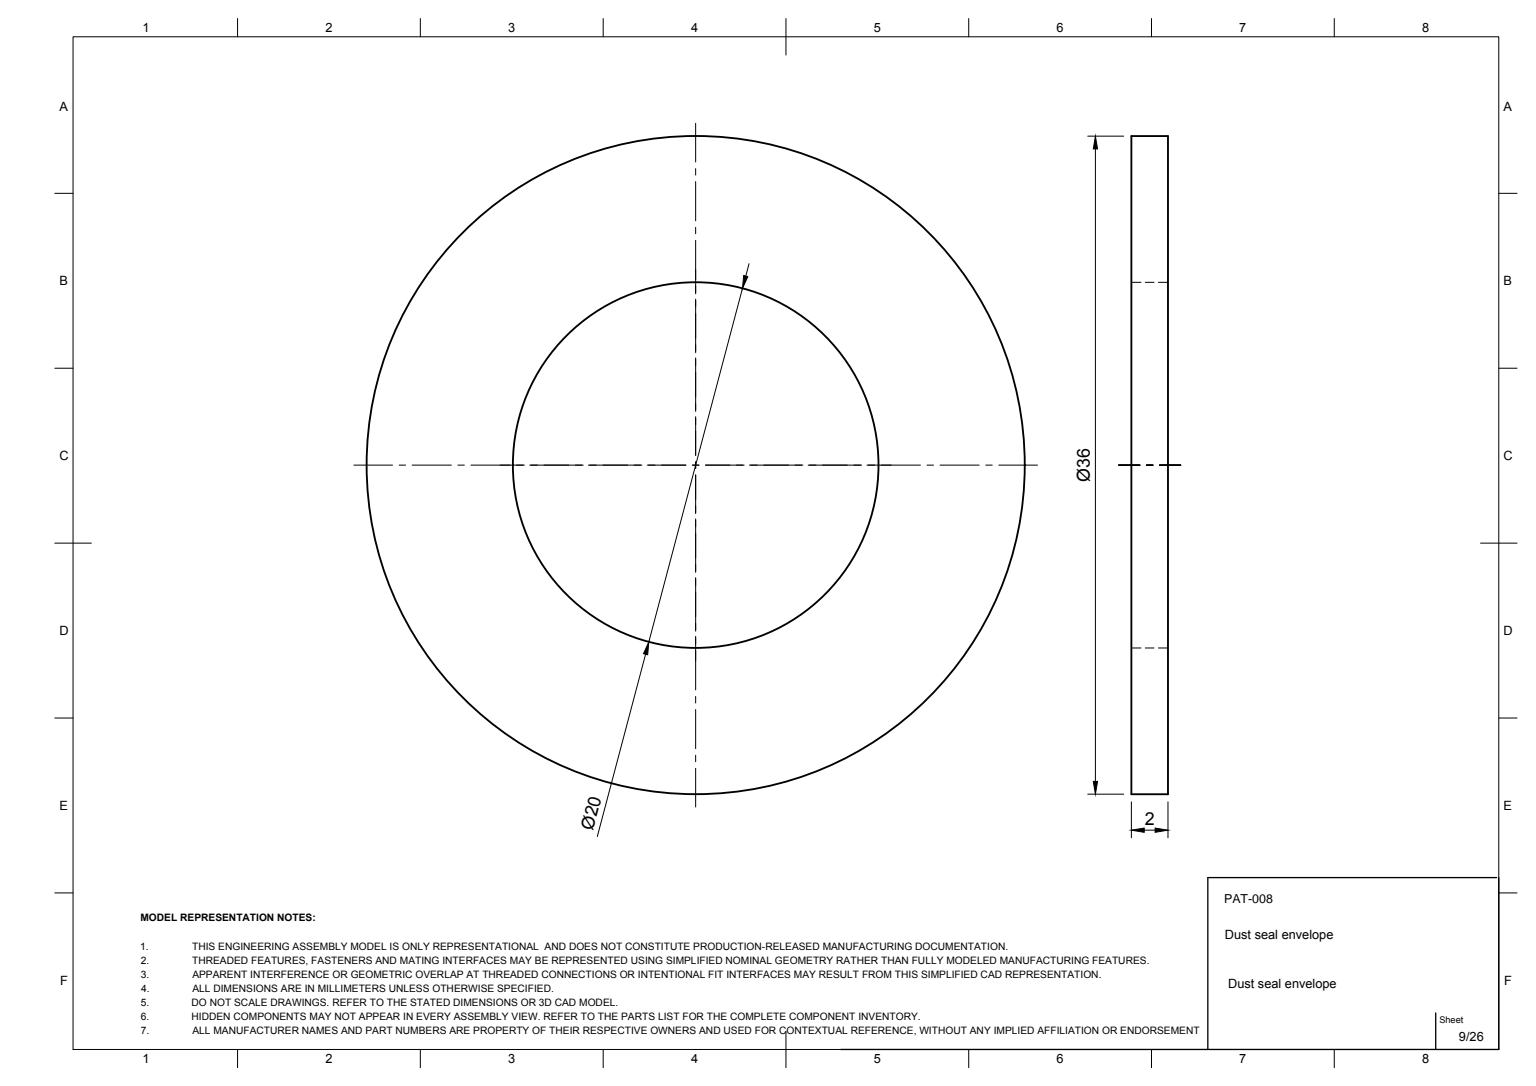
ISO-10303-21;
HEADER;
/* Generated by software containing ST-Developer
 * from STEP Tools, Inc. (www.steptools.com) 
 */

FILE_DESCRIPTION(
/* description */ ('Bearing housing with oil seal and end cap'),
/* implementation_level */ '2;1');

FILE_NAME(
/* name */ 'Dust seal envelope.step',
/* time_stamp */ '2026-10-28T03:23:10-07:00',
/* author */ (''),
/* organization */ (''),
/* preprocessor_version */ 'ST-DEVELOPER v20.2',
/* originating_system */ 'Autodesk Translation Framework v15.17.0.0',
/* authorisation */ '');

FILE_SCHEMA (('AUTOMOTIVE_DESIGN { 1 0 10303 214 3 1 1 }'));
ENDSEC;

DATA;
#10=MECHANICAL_DESIGN_GEOMETRIC_PRESENTATION_REPRESENTATION('',(#263),#7871);
#221=SHAPE_REPRESENTATION_RELATIONSHIP('SRR','None',#7968,#242);
#242=ADVANCED_BREP_SHAPE_REPRESENTATION('',(#292),#7852);
#263=STYLED_ITEM('',(#8160),#292);
#292=MANIFOLD_SOLID_BREP('Body1',#4089);
#357=FACE_BOUND('',#916,.T.);
#358=FACE_BOUND('',#918,.T.);
#448=PLANE('',#4493);
#449=PLANE('',#4494);
#620=FACE_OUTER_BOUND('',#913,.T.);
#621=FACE_OUTER_BOUND('',#914,.T.);
#622=FACE_OUTER_BOUND('',#915,.T.);
#623=FACE_OUTER_BOUND('',#917,.T.);
#913=EDGE_LOOP('',(#3023,#3024,#3025,#3026));
#914=EDGE_LOOP('',(#3027,#3028,#3029,#3030));
#915=EDGE_LOOP('',(#3031));
#916=EDGE_LOOP('',(#3032));
#917=EDGE_LOOP('',(#3033));
#918=EDGE_LOOP('',(#3034));
#1223=LINE('',#6517,#1485);
#1224=LINE('',#6523,#1486);
#1485=VECTOR('',#5238,1.);
#1486=VECTOR('',#5245,1.8);
#1735=CIRCLE('',#4488,1.);
#1736=CIRCLE('',#4489,1.);
#1737=CIRCLE('',#4491,1.8);
#1738=CIRCLE('',#4492,1.8);
#1983=VERTEX_POINT('',#6514);
#1984=VERTEX_POINT('',#6516);
#1985=VERTEX_POINT('',#6520);
#1986=VERTEX_POINT('',#6522);
#2375=EDGE_CURVE('',#1983,#1983,#1735,.T.);
#2376=EDGE_CURVE('',#1983,#1984,#1223,.T.);
#2377=EDGE_CURVE('',#1984,#1984,#1736,.T.);
#2378=EDGE_CURVE('',#1985,#1985,#1737,.T.);
#2379=EDGE_CURVE('',#1985,#1986,#1224,.T.);
#2380=EDGE_CURVE('',#1986,#1986,#1738,.T.);
#3023=ORIENTED_EDGE('',*,*,#2375,.F.);
#3024=ORIENTED_EDGE('',*,*,#2376,.T.);
#3025=ORIENTED_EDGE('',*,*,#2377,.T.);
#3026=ORIENTED_EDGE('',*,*,#2376,.F.);
#3027=ORIENTED_EDGE('',*,*,#2378,.F.);
#3028=ORIENTED_EDGE('',*,*,#2379,.T.);
#3029=ORIENTED_EDGE('',*,*,#2380,.T.);
#3030=ORIENTED_EDGE('',*,*,#2379,.F.);
#3031=ORIENTED_EDGE('',*,*,#2378,.T.);
#3032=ORIENTED_EDGE('',*,*,#2375,.T.);
#3033=ORIENTED_EDGE('',*,*,#2380,.F.);
#3034=ORIENTED_EDGE('',*,*,#2377,.F.);
#3787=CYLINDRICAL_SURFACE('',#4487,1.);
#3788=CYLINDRICAL_SURFACE('',#4490,1.8);
#3902=ADVANCED_FACE('',(#620),#3787,.F.);
#3903=ADVANCED_FACE('',(#621),#3788,.T.);
#3904=ADVANCED_FACE('',(#622,#357),#448,.T.);
#3905=ADVANCED_FACE('',(#623,#358),#449,.F.);
#4089=CLOSED_SHELL('',(#3902,#3903,#3904,#3905));
#4486=AXIS2_PLACEMENT_3D('',#6512,#5232,#5233);
#4487=AXIS2_PLACEMENT_3D('',#6513,#5234,#5235);
#4488=AXIS2_PLACEMENT_3D('',#6515,#5236,#5237);
#4489=AXIS2_PLACEMENT_3D('',#6518,#5239,#5240);
#4490=AXIS2_PLACEMENT_3D('',#6519,#5241,#5242);
#4491=AXIS2_PLACEMENT_3D('',#6521,#5243,#5244);
#4492=AXIS2_PLACEMENT_3D('',#6524,#5246,#5247);
#4493=AXIS2_PLACEMENT_3D('',#6525,#5248,#5249);
#4494=AXIS2_PLACEMENT_3D('',#6526,#5250,#5251);
#5232=DIRECTION('axis',(0.,0.,1.));
#5233=DIRECTION('refdir',(1.,0.,0.));
#5234=DIRECTION('center_axis',(0.,1.,0.));
#5235=DIRECTION('ref_axis',(1.,0.,0.));
#5236=DIRECTION('center_axis',(0.,-1.,0.));
#5237=DIRECTION('ref_axis',(1.,0.,0.));
#5238=DIRECTION('',(0.,-1.,0.));
#5239=DIRECTION('center_axis',(0.,-1.,0.));
#5240=DIRECTION('ref_axis',(1.,0.,0.));
#5241=DIRECTION('center_axis',(0.,1.,0.));
#5242=DIRECTION('ref_axis',(1.,0.,0.));
#5243=DIRECTION('center_axis',(0.,1.,0.));
#5244=DIRECTION('ref_axis',(1.,0.,0.));
#5245=DIRECTION('',(0.,-1.,0.));
#5246=DIRECTION('center_axis',(0.,1.,0.));
#5247=DIRECTION('ref_axis',(1.,0.,0.));
#5248=DIRECTION('center_axis',(0.,1.,0.));
#5249=DIRECTION('ref_axis',(1.,0.,0.));
#5250=DIRECTION('center_axis',(0.,1.,0.));
#5251=DIRECTION('ref_axis',(1.,0.,0.));
#6512=CARTESIAN_POINT('',(0.,0.,0.));
#6513=CARTESIAN_POINT('Origin',(0.,-0.4,4.5));
#6514=CARTESIAN_POINT('',(-1.,-0.2,4.5));
#6515=CARTESIAN_POINT('Origin',(0.,-0.2,4.5));
#6516=CARTESIAN_POINT('',(-1.,-0.4,4.5));
#6517=CARTESIAN_POINT('',(-1.,-0.4,4.5));
#6518=CARTESIAN_POINT('Origin',(0.,-0.4,4.5));
#6519=CARTESIAN_POINT('Origin',(0.,-0.4,4.5));
#6520=CARTESIAN_POINT('',(-1.8,-0.2,4.5));
#6521=CARTESIAN_POINT('Origin',(0.,-0.2,4.5));
#6522=CARTESIAN_POINT('',(-1.8,-0.4,4.5));
#6523=CARTESIAN_POINT('',(-1.8,-0.4,4.5));
#6524=CARTESIAN_POINT('Origin',(0.,-0.4,4.5));
#6525=CARTESIAN_POINT('Origin',(0.,-0.2,4.5));
#6526=CARTESIAN_POINT('Origin',(0.,-0.4,4.5));
#7826=UNCERTAINTY_MEASURE_WITH_UNIT(LENGTH_MEASURE(0.001),#7872,
'DISTANCE_ACCURACY_VALUE',
'Maximum model space distance between geometric entities at asserted c
onnectivities');
#7845=UNCERTAINTY_MEASURE_WITH_UNIT(LENGTH_MEASURE(0.001),#7872,
'DISTANCE_ACCURACY_VALUE',
'Maximum model space distance between geometric entities at asserted c
onnectivities');
#7852=(
GEOMETRIC_REPRESENTATION_CONTEXT(3)
GLOBAL_UNCERTAINTY_ASSIGNED_CONTEXT((#7826))
GLOBAL_UNIT_ASSIGNED_CONTEXT((#7872,#7874,#7875))
REPRESENTATION_CONTEXT('','3D')
);
#7871=(
GEOMETRIC_REPRESENTATION_CONTEXT(3)
GLOBAL_UNCERTAINTY_ASSIGNED_CONTEXT((#7845))
GLOBAL_UNIT_ASSIGNED_CONTEXT((#7872,#7874,#7875))
REPRESENTATION_CONTEXT('','3D')
);
#7872=(
LENGTH_UNIT()
NAMED_UNIT(*)
SI_UNIT(.CENTI.,.METRE.)
);
#7874=(
NAMED_UNIT(*)
PLANE_ANGLE_UNIT()
SI_UNIT($,.RADIAN.)
);
#7875=(
NAMED_UNIT(*)
SI_UNIT($,.STERADIAN.)
SOLID_ANGLE_UNIT()
);
#7882=SHAPE_DEFINITION_REPRESENTATION(#7907,#7968);
#7907=PRODUCT_DEFINITION_SHAPE('',$,#7994);
#7968=SHAPE_REPRESENTATION('',(#4486),#7852);
#7987=PRODUCT_DEFINITION_CONTEXT('part definition',#8064,'design');
#7994=PRODUCT_DEFINITION('Dust seal envelope','Dust seal envelope',#8019,
#7987);
#8019=PRODUCT_DEFINITION_FORMATION('',$,#8072);
#8064=APPLICATION_CONTEXT(
'Core Data for Automotive Mechanical Design Process');
#8065=PRODUCT_CONTEXT('part definition',#8064,'mechanical');
#8072=PRODUCT('Dust seal envelope','Dust seal envelope',
'Dust seal envelope',(#8065));
#8154=COLOUR_RGB('Black',0.12,0.14,0.17);
#8155=FILL_AREA_STYLE_COLOUR('',#8154);
#8156=FILL_AREA_STYLE('',(#8155));
#8157=SURFACE_STYLE_FILL_AREA(#8156);
#8158=SURFACE_SIDE_STYLE('',(#8157));
#8159=SURFACE_STYLE_USAGE(.BOTH.,#8158);
#8160=PRESENTATION_STYLE_ASSIGNMENT((#8159));
ENDSEC;
END-ISO-10303-21;
